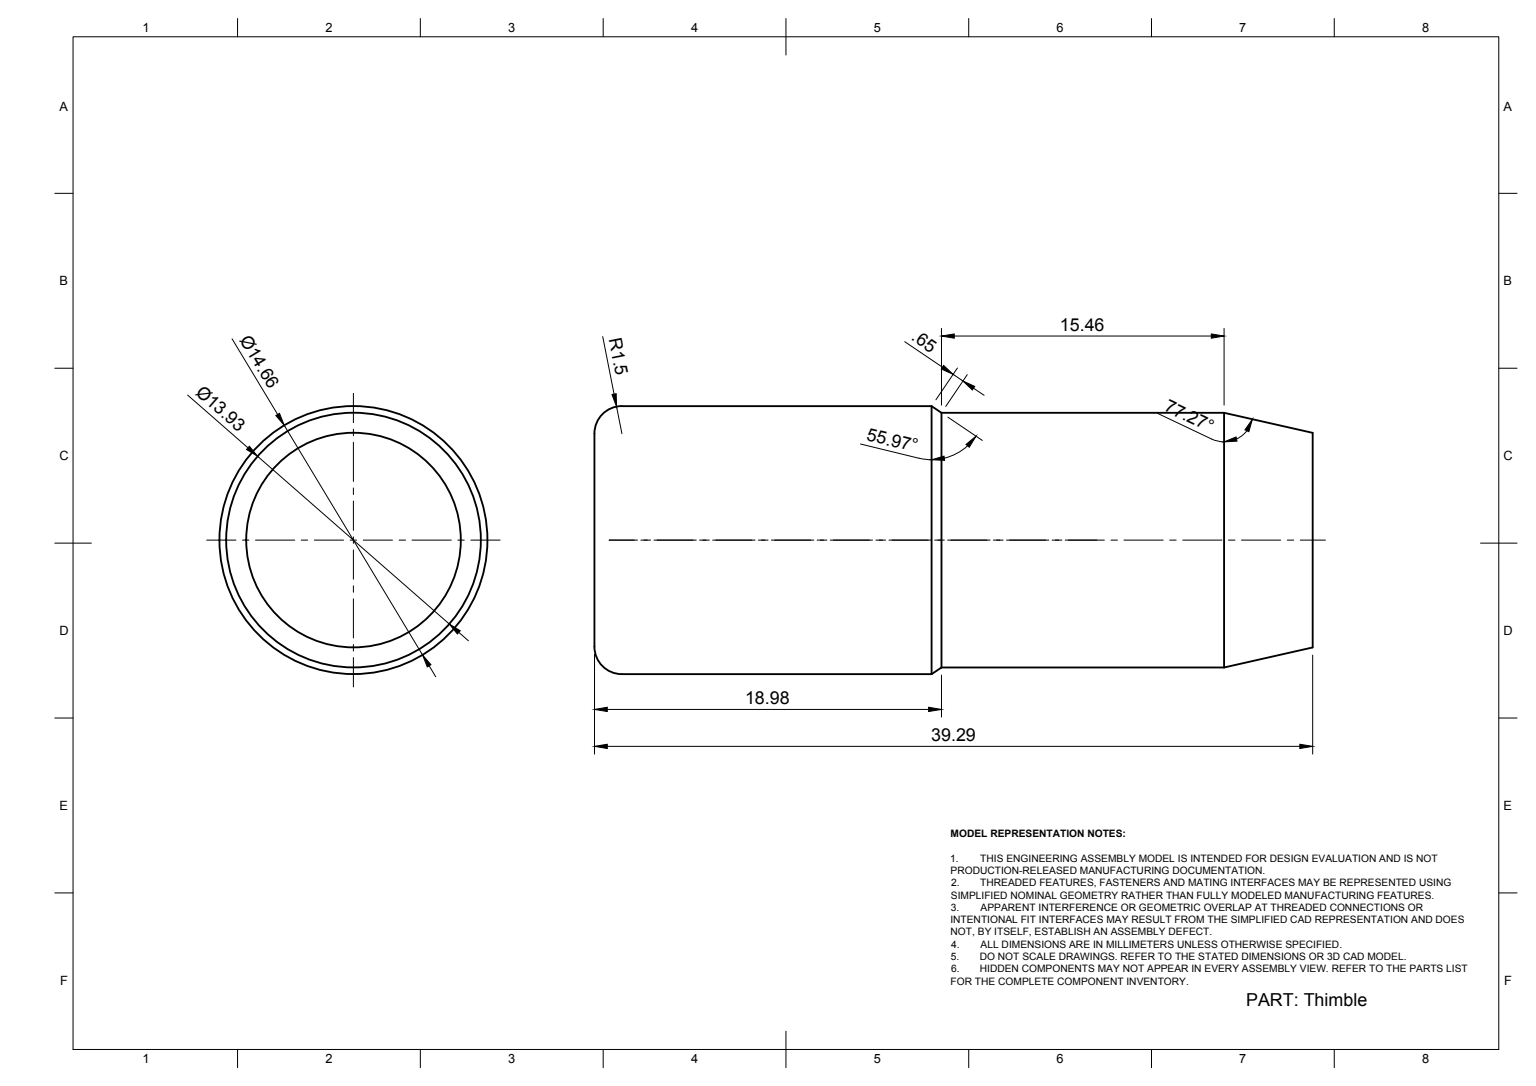
ISO-10303-21;
HEADER;
/* Generated by software containing ST-Developer
 * from STEP Tools, Inc. (www.steptools.com) 
 */

FILE_DESCRIPTION(
/* description */ (''),
/* implementation_level */ '2;1');

FILE_NAME(
/* name */ 'Thimble.step',
/* time_stamp */ '2026-10-05T01:33:24-07:00',
/* author */ (''),
/* organization */ (''),
/* preprocessor_version */ 'ST-DEVELOPER v20.2',
/* originating_system */ 'Autodesk Translation Framework v15.15.0.0',
/* authorisation */ '');

FILE_SCHEMA (('AUTOMOTIVE_DESIGN { 1 0 10303 214 3 1 1 }'));
ENDSEC;

DATA;
#10=MECHANICAL_DESIGN_GEOMETRIC_PRESENTATION_REPRESENTATION('',(#83),#1128);
#51=TOROIDAL_SURFACE('',#659,5.82799886529799,1.5);
#55=CONICAL_SURFACE('',#650,6.41661225190487,0.22222982204112);
#56=CONICAL_SURFACE('',#655,7.14605510547863,0.59398290857058);
#63=SHAPE_REPRESENTATION_RELATIONSHIP('SRR','None',#1167,#73);
#73=ADVANCED_BREP_SHAPE_REPRESENTATION('',(#93),#1119);
#83=STYLED_ITEM('',(#1225),#93);
#93=MANIFOLD_SOLID_BREP('Body1',#522);
#103=LINE('',#971,#120);
#104=LINE('',#976,#121);
#105=LINE('',#980,#122);
#106=LINE('',#984,#123);
#120=VECTOR('',#762,6.41661225190487);
#121=VECTOR('',#769,6.96411134565927);
#122=VECTOR('',#774,7.14605510547863);
#123=VECTOR('',#779,7.327998865298);
#137=CYLINDRICAL_SURFACE('',#653,6.96411134565927);
#138=CYLINDRICAL_SURFACE('',#657,7.327998865298);
#149=FACE_OUTER_BOUND('',#190,.T.);
#150=FACE_OUTER_BOUND('',#191,.T.);
#151=FACE_OUTER_BOUND('',#192,.T.);
#152=FACE_OUTER_BOUND('',#193,.T.);
#153=FACE_OUTER_BOUND('',#194,.T.);
#154=FACE_OUTER_BOUND('',#195,.T.);
#155=FACE_OUTER_BOUND('',#196,.T.);
#190=EDGE_LOOP('',(#358,#359,#360,#361));
#191=EDGE_LOOP('',(#362,#363,#364,#365));
#192=EDGE_LOOP('',(#366,#367,#368,#369));
#193=EDGE_LOOP('',(#370,#371,#372,#373));
#194=EDGE_LOOP('',(#374,#375,#376,#377));
#195=EDGE_LOOP('',(#378));
#196=EDGE_LOOP('',(#379));
#230=CIRCLE('',#651,6.96411134565927);
#231=CIRCLE('',#652,5.86911315815046);
#232=CIRCLE('',#654,6.96411134565926);
#233=CIRCLE('',#656,7.327998865298);
#234=CIRCLE('',#658,7.327998865298);
#235=CIRCLE('',#660,5.827998865298);
#236=CIRCLE('',#661,1.5);
#267=VERTEX_POINT('',#968);
#268=VERTEX_POINT('',#970);
#269=VERTEX_POINT('',#974);
#270=VERTEX_POINT('',#978);
#271=VERTEX_POINT('',#982);
#272=VERTEX_POINT('',#986);
#301=EDGE_CURVE('',#267,#267,#230,.T.);
#302=EDGE_CURVE('',#267,#268,#103,.T.);
#303=EDGE_CURVE('',#268,#268,#231,.T.);
#304=EDGE_CURVE('',#269,#269,#232,.T.);
#305=EDGE_CURVE('',#269,#267,#104,.T.);
#306=EDGE_CURVE('',#270,#270,#233,.T.);
#307=EDGE_CURVE('',#270,#269,#105,.T.);
#308=EDGE_CURVE('',#271,#271,#234,.T.);
#309=EDGE_CURVE('',#271,#270,#106,.T.);
#310=EDGE_CURVE('',#272,#272,#235,.T.);
#311=EDGE_CURVE('',#272,#271,#236,.T.);
#358=ORIENTED_EDGE('',*,*,#301,.F.);
#359=ORIENTED_EDGE('',*,*,#302,.T.);
#360=ORIENTED_EDGE('',*,*,#303,.T.);
#361=ORIENTED_EDGE('',*,*,#302,.F.);
#362=ORIENTED_EDGE('',*,*,#304,.F.);
#363=ORIENTED_EDGE('',*,*,#305,.T.);
#364=ORIENTED_EDGE('',*,*,#301,.T.);
#365=ORIENTED_EDGE('',*,*,#305,.F.);
#366=ORIENTED_EDGE('',*,*,#306,.F.);
#367=ORIENTED_EDGE('',*,*,#307,.T.);
#368=ORIENTED_EDGE('',*,*,#304,.T.);
#369=ORIENTED_EDGE('',*,*,#307,.F.);
#370=ORIENTED_EDGE('',*,*,#308,.F.);
#371=ORIENTED_EDGE('',*,*,#309,.T.);
#372=ORIENTED_EDGE('',*,*,#306,.T.);
#373=ORIENTED_EDGE('',*,*,#309,.F.);
#374=ORIENTED_EDGE('',*,*,#310,.F.);
#375=ORIENTED_EDGE('',*,*,#311,.T.);
#376=ORIENTED_EDGE('',*,*,#308,.T.);
#377=ORIENTED_EDGE('',*,*,#311,.F.);
#378=ORIENTED_EDGE('',*,*,#310,.T.);
#379=ORIENTED_EDGE('',*,*,#303,.F.);
#462=PLANE('',#662);
#463=PLANE('',#663);
#483=ADVANCED_FACE('',(#149),#55,.T.);
#484=ADVANCED_FACE('',(#150),#137,.T.);
#485=ADVANCED_FACE('',(#151),#56,.T.);
#486=ADVANCED_FACE('',(#152),#138,.T.);
#487=ADVANCED_FACE('',(#153),#51,.T.);
#488=ADVANCED_FACE('',(#154),#462,.T.);
#489=ADVANCED_FACE('',(#155),#463,.T.);
#522=CLOSED_SHELL('',(#483,#484,#485,#486,#487,#488,#489));
#649=AXIS2_PLACEMENT_3D('',#966,#756,#757);
#650=AXIS2_PLACEMENT_3D('',#967,#758,#759);
#651=AXIS2_PLACEMENT_3D('',#969,#760,#761);
#652=AXIS2_PLACEMENT_3D('',#972,#763,#764);
#653=AXIS2_PLACEMENT_3D('',#973,#765,#766);
#654=AXIS2_PLACEMENT_3D('',#975,#767,#768);
#655=AXIS2_PLACEMENT_3D('',#977,#770,#771);
#656=AXIS2_PLACEMENT_3D('',#979,#772,#773);
#657=AXIS2_PLACEMENT_3D('',#981,#775,#776);
#658=AXIS2_PLACEMENT_3D('',#983,#777,#778);
#659=AXIS2_PLACEMENT_3D('',#985,#780,#781);
#660=AXIS2_PLACEMENT_3D('',#987,#782,#783);
#661=AXIS2_PLACEMENT_3D('',#988,#784,#785);
#662=AXIS2_PLACEMENT_3D('',#989,#786,#787);
#663=AXIS2_PLACEMENT_3D('',#990,#788,#789);
#756=DIRECTION('axis',(0.,0.,1.));
#757=DIRECTION('refdir',(1.,0.,0.));
#758=DIRECTION('center_axis',(1.,0.,0.));
#759=DIRECTION('ref_axis',(0.,0.,-1.));
#760=DIRECTION('center_axis',(1.,0.,0.));
#761=DIRECTION('ref_axis',(0.,0.,-1.));
#762=DIRECTION('',(-0.975408410378343,2.69918469288288E-17,-0.220405156389757));
#763=DIRECTION('center_axis',(1.,0.,0.));
#764=DIRECTION('ref_axis',(0.,0.,-1.));
#765=DIRECTION('center_axis',(1.,0.,0.));
#766=DIRECTION('ref_axis',(0.,0.,-1.));
#767=DIRECTION('center_axis',(1.,0.,0.));
#768=DIRECTION('ref_axis',(0.,0.,-1.));
#769=DIRECTION('',(-1.,0.,0.));
#770=DIRECTION('center_axis',(1.,0.,0.));
#771=DIRECTION('ref_axis',(0.,0.,-1.));
#772=DIRECTION('center_axis',(1.,0.,0.));
#773=DIRECTION('ref_axis',(0.,0.,-1.));
#774=DIRECTION('',(-0.828718159042203,6.85393373868948E-17,-0.559666161987396));
#775=DIRECTION('center_axis',(1.,0.,0.));
#776=DIRECTION('ref_axis',(0.,0.,-1.));
#777=DIRECTION('center_axis',(1.,0.,0.));
#778=DIRECTION('ref_axis',(0.,0.,-1.));
#779=DIRECTION('',(-1.,0.,0.));
#780=DIRECTION('center_axis',(1.,0.,0.));
#781=DIRECTION('ref_axis',(0.,0.,-1.));
#782=DIRECTION('center_axis',(1.,0.,0.));
#783=DIRECTION('ref_axis',(0.,0.,-1.));
#784=DIRECTION('center_axis',(0.,-1.,-1.22464679914735E-16));
#785=DIRECTION('ref_axis',(0.,-1.22464679914735E-16,1.));
#786=DIRECTION('center_axis',(1.,0.,0.));
#787=DIRECTION('ref_axis',(0.,0.,-1.));
#788=DIRECTION('center_axis',(-1.,0.,0.));
#789=DIRECTION('ref_axis',(0.,0.,1.));
#966=CARTESIAN_POINT('',(0.,0.,0.));
#967=CARTESIAN_POINT('Origin',(49.7315453550068,0.,0.));
#968=CARTESIAN_POINT('',(52.1545159854134,-8.52857666836739E-16,6.96411134565927));
#969=CARTESIAN_POINT('Origin',(52.1545159854134,0.,0.));
#970=CARTESIAN_POINT('',(47.3085747246001,-7.18759064296257E-16,5.86911315815046));
#971=CARTESIAN_POINT('',(49.7315453550068,-7.85808365566499E-16,6.41661225190487));
#972=CARTESIAN_POINT('Origin',(47.3085747246001,0.,0.));
#973=CARTESIAN_POINT('Origin',(59.8855873271505,0.,0.));
#974=CARTESIAN_POINT('',(67.6166586688876,-8.52857666836739E-16,6.96411134565927));
#975=CARTESIAN_POINT('Origin',(67.6166586688876,0.,0.));
#976=CARTESIAN_POINT('',(59.8855873271505,-8.52857666836739E-16,6.96411134565927));
#977=CARTESIAN_POINT('Origin',(67.8860694496847,0.,0.));
#978=CARTESIAN_POINT('',(68.1554802304818,-8.97421035454263E-16,7.327998865298));
#979=CARTESIAN_POINT('Origin',(68.1554802304818,0.,0.));
#980=CARTESIAN_POINT('',(67.8860694496847,-8.75139351145501E-16,7.14605510547863));
#981=CARTESIAN_POINT('Origin',(76.6276350483148,0.,0.));
#982=CARTESIAN_POINT('',(85.0997898661478,-8.97421035454263E-16,7.327998865298));
#983=CARTESIAN_POINT('Origin',(85.0997898661478,0.,0.));
#984=CARTESIAN_POINT('',(76.6276350483148,-8.97421035454263E-16,7.327998865298));
#985=CARTESIAN_POINT('Origin',(85.0997898661478,0.,0.));
#986=CARTESIAN_POINT('',(86.5997898661478,-7.1372401558216E-16,5.827998865298));
#987=CARTESIAN_POINT('Origin',(86.5997898661478,0.,0.));
#988=CARTESIAN_POINT('Origin',(85.0997898661478,-7.13724015582159E-16,5.82799886529799));
#989=CARTESIAN_POINT('Origin',(86.5997898661478,0.,0.));
#990=CARTESIAN_POINT('Origin',(47.3085747246001,0.,-5.86911315815046));
#1107=UNCERTAINTY_MEASURE_WITH_UNIT(LENGTH_MEASURE(0.01),#1129,
'DISTANCE_ACCURACY_VALUE',
'Maximum model space distance between geometric entities at asserted c
onnectivities');
#1116=UNCERTAINTY_MEASURE_WITH_UNIT(LENGTH_MEASURE(0.01),#1129,
'DISTANCE_ACCURACY_VALUE',
'Maximum model space distance between geometric entities at asserted c
onnectivities');
#1119=(
GEOMETRIC_REPRESENTATION_CONTEXT(3)
GLOBAL_UNCERTAINTY_ASSIGNED_CONTEXT((#1107))
GLOBAL_UNIT_ASSIGNED_CONTEXT((#1129,#1131,#1132))
REPRESENTATION_CONTEXT('','3D')
);
#1128=(
GEOMETRIC_REPRESENTATION_CONTEXT(3)
GLOBAL_UNCERTAINTY_ASSIGNED_CONTEXT((#1116))
GLOBAL_UNIT_ASSIGNED_CONTEXT((#1129,#1131,#1132))
REPRESENTATION_CONTEXT('','3D')
);
#1129=(
LENGTH_UNIT()
NAMED_UNIT(*)
SI_UNIT(.MILLI.,.METRE.)
);
#1131=(
NAMED_UNIT(*)
PLANE_ANGLE_UNIT()
SI_UNIT($,.RADIAN.)
);
#1132=(
NAMED_UNIT(*)
SI_UNIT($,.STERADIAN.)
SOLID_ANGLE_UNIT()
);
#1135=SHAPE_DEFINITION_REPRESENTATION(#1146,#1167);
#1146=PRODUCT_DEFINITION_SHAPE('',$,#1179);
#1167=SHAPE_REPRESENTATION('',(#649),#1119);
#1176=PRODUCT_DEFINITION_CONTEXT('part definition',#1211,'design');
#1179=PRODUCT_DEFINITION('Thimble','Thimble',#1190,#1176);
#1190=PRODUCT_DEFINITION_FORMATION('',$,#1215);
#1211=APPLICATION_CONTEXT(
'Core Data for Automotive Mechanical Design Process');
#1212=PRODUCT_CONTEXT('part definition',#1211,'mechanical');
#1215=PRODUCT('Thimble','Thimble',$,(#1212));
#1225=PRESENTATION_STYLE_ASSIGNMENT((#1229));
#1229=SURFACE_STYLE_USAGE(.BOTH.,#1233);
#1233=SURFACE_SIDE_STYLE('',(#1237));
#1237=SURFACE_STYLE_FILL_AREA(#1241);
#1241=FILL_AREA_STYLE('Opaque(201,201,201)',(#1245));
#1245=FILL_AREA_STYLE_COLOUR('Opaque(201,201,201)',#1249);
#1249=COLOUR_RGB('Opaque(201,201,201)', 0.09019608, 0.27058824, 0.51372549);
ENDSEC;
END-ISO-10303-21;
